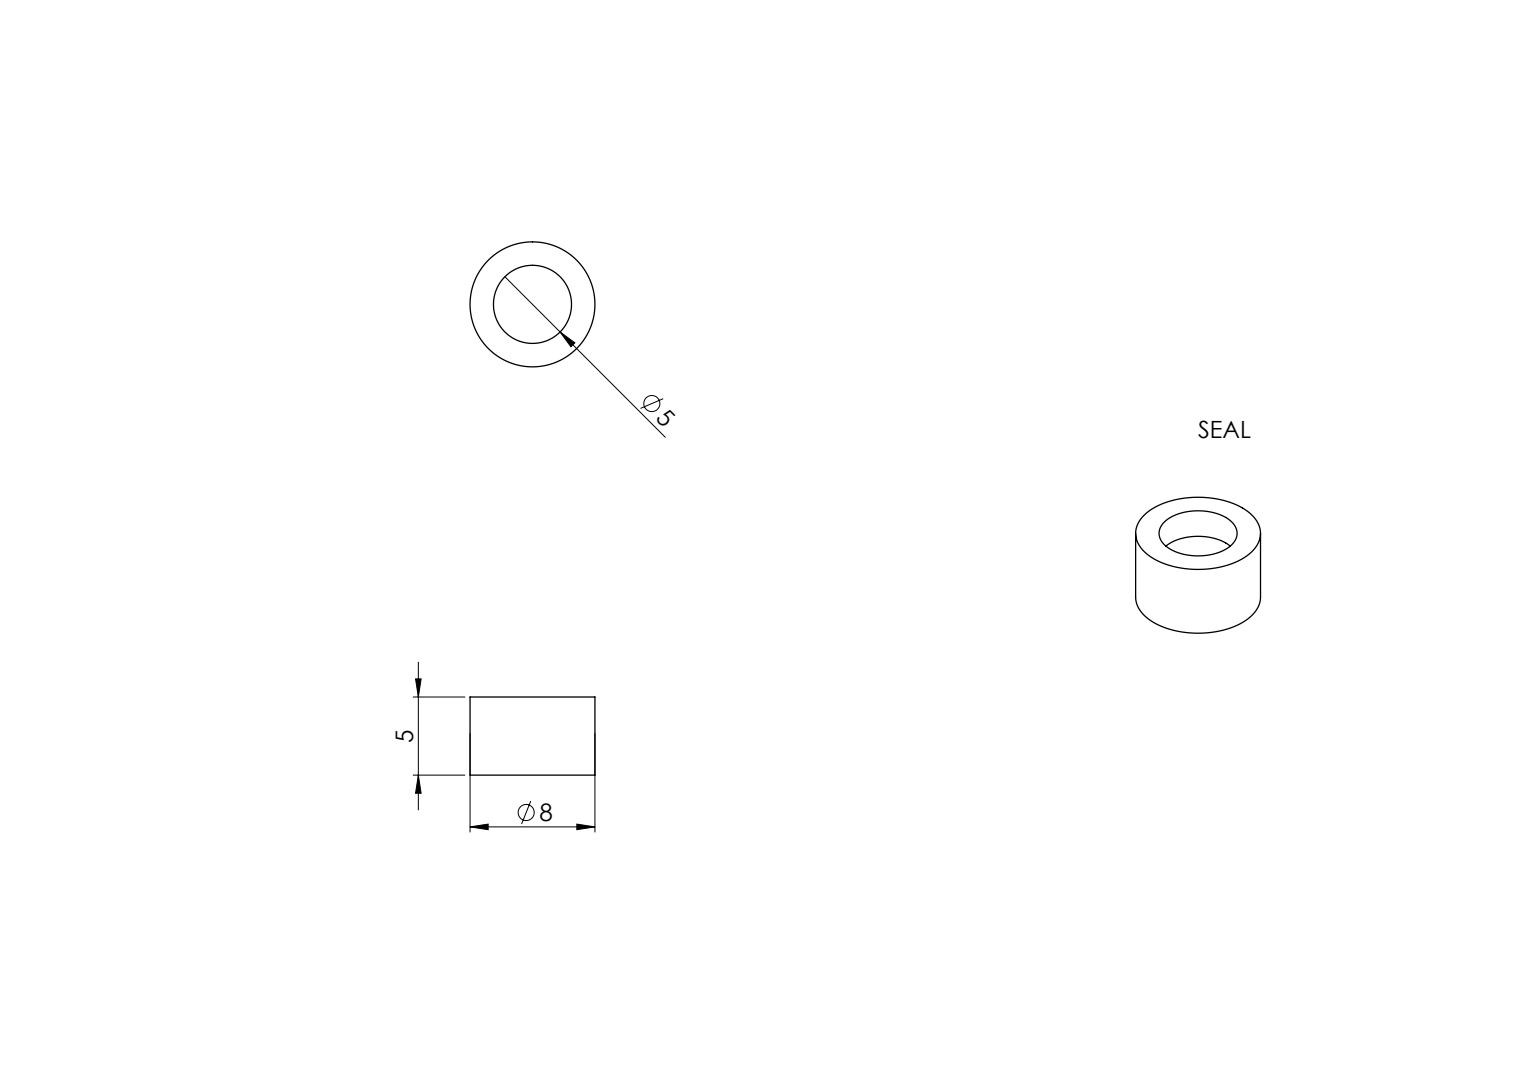
ISO-10303-21;
HEADER;
FILE_DESCRIPTION (('STEP AP214'),
    '1' );
FILE_NAME ('seal.step',
    '2026-10-25T16:39:07',
    ( '' ),
    ( '' ),
    'SwSTEP 2.0',
    'SolidWorks 2026',
    '' );
FILE_SCHEMA (( 'AUTOMOTIVE_DESIGN' ));
ENDSEC;

DATA;
#4=CIRCLE ( 'NONE', #8561, 2.499999999999999556 ) ;
#17=CARTESIAN_POINT ( 'NONE',  ( 0.000000000000000000, 0.000000000000000000, 4.000000000000000000 ) ) ;
#234=CARTESIAN_POINT ( 'NONE',  ( 3.061616997868382648E-16, 3.000000000000000000, -2.499999999999999556 ) ) ;
#340=( GEOMETRIC_REPRESENTATION_CONTEXT ( 3 ) GLOBAL_UNCERTAINTY_ASSIGNED_CONTEXT ( ( #12516 ) ) GLOBAL_UNIT_ASSIGNED_CONTEXT ( ( #1395, #8421, #14269 ) ) REPRESENTATION_CONTEXT ( 'NONE', 'WORKASPACE' ) );
#392=DIRECTION ( 'NONE',  ( 0.000000000000000000, -1.000000000000000000, 0.000000000000000000 ) ) ;
#724=VECTOR ( 'NONE', #10694, 1000.000000000000000 ) ;
#725=PRODUCT_DEFINITION_SHAPE ( 'NONE', 'NONE',  #2104 ) ;
#866=ORIENTED_EDGE ( 'NONE', *, *, #16394, .T. ) ;
#914=AXIS2_PLACEMENT_3D ( 'NONE', #3726, #9376, #2718 ) ;
#1063=DIRECTION ( 'NONE',  ( 0.000000000000000000, -1.000000000000000000, 0.000000000000000000 ) ) ;
#1236=ORIENTED_EDGE ( 'NONE', *, *, #16460, .F. ) ;
#1279=CARTESIAN_POINT ( 'NONE',  ( 0.000000000000000000, 3.000000000000000000, 0.000000000000000000 ) ) ;
#1296=AXIS2_PLACEMENT_3D ( 'NONE', #7926, #9407, #3852 ) ;
#1381=EDGE_CURVE ( 'NONE', #5033, #1782, #14887, .T. ) ;
#1393=FACE_OUTER_BOUND ( 'NONE', #4236, .T. ) ;
#1395=( LENGTH_UNIT ( ) NAMED_UNIT ( * ) SI_UNIT ( .MILLI., .METRE. ) );
#1483=( LENGTH_UNIT ( ) NAMED_UNIT ( * ) SI_UNIT ( .MILLI., .METRE. ) );
#1500=VERTEX_POINT ( 'NONE', #13446 ) ;
#1507=AXIS2_PLACEMENT_3D ( 'NONE', #2357, #6777, #8078 ) ;
#1556=PRODUCT_DEFINITION_FORMATION_WITH_SPECIFIED_SOURCE ( 'ANY', '', #17623, .NOT_KNOWN. ) ;
#1572=PLANE ( 'NONE',  #2737 ) ;
#1586=MANIFOLD_SOLID_BREP ( 'Boss-Extrude2', #14466 ) ;
#1614=CYLINDRICAL_SURFACE ( 'NONE', #16233, 2.499999999999999556 ) ;
#1655=ORIENTED_EDGE ( 'NONE', *, *, #16460, .T. ) ;
#1782=VERTEX_POINT ( 'NONE', #10171 ) ;
#1803=ORIENTED_EDGE ( 'NONE', *, *, #5917, .F. ) ;
#1935=CARTESIAN_POINT ( 'NONE',  ( 0.000000000000000000, 5.000000000000000000, 2.499999999999999556 ) ) ;
#2104=PRODUCT_DEFINITION ( 'UNKNOWN', '', #1556, #14150 ) ;
#2168=STYLED_ITEM('',(#18417),#1586);
#2227=VERTEX_POINT ( 'NONE', #17 ) ;
#2331=LINE ( 'NONE', #12225, #8909 ) ;
#2357=CARTESIAN_POINT ( 'NONE',  ( 0.000000000000000000, 5.000000000000000000, 0.000000000000000000 ) ) ;
#2461=FILL_AREA_STYLE_COLOUR ( '', #10696 ) ;
#2511=ORIENTED_EDGE ( 'NONE', *, *, #16394, .F. ) ;
#2541=CARTESIAN_POINT ( 'NONE',  ( 4.898587196589414801E-16, 0.000000000000000000, -4.000000000000000000 ) ) ;
#2624=DIRECTION ( 'NONE',  ( 0.000000000000000000, 0.000000000000000000, 1.000000000000000000 ) ) ;
#2711=ORIENTED_EDGE ( 'NONE', *, *, #4160, .F. ) ;
#2717=STYLED_ITEM ( 'NONE', ( #12687 ), #5178 ) ;
#2718=DIRECTION ( 'NONE',  ( 0.000000000000000000, 0.000000000000000000, 1.000000000000000000 ) ) ;
#2737=AXIS2_PLACEMENT_3D ( 'NONE', #11659, #7020, #14460 ) ;
#2801=DIRECTION ( 'NONE',  ( 0.000000000000000000, 0.000000000000000000, -1.000000000000000000 ) ) ;
#2957=AXIS2_PLACEMENT_3D ( 'NONE', #8286, #17957, #5417 ) ;
#3271=ADVANCED_FACE ( 'NONE', ( #1393, #15571 ), #1572, .F. ) ;
#3674=DIRECTION ( 'NONE',  ( -0.000000000000000000, 1.000000000000000000, -0.000000000000000000 ) ) ;
#3726=CARTESIAN_POINT ( 'NONE',  ( 0.000000000000000000, 3.000000000000000000, 0.000000000000000000 ) ) ;
#3852=DIRECTION ( 'NONE',  ( 0.000000000000000000, -0.000000000000000000, -1.000000000000000000 ) ) ;
#3895=( LENGTH_UNIT ( ) NAMED_UNIT ( * ) SI_UNIT ( .MILLI., .METRE. ) );
#4160=EDGE_CURVE ( 'NONE', #9997, #1782, #12097, .T. ) ;
#4200=MECHANICAL_DESIGN_GEOMETRIC_PRESENTATION_REPRESENTATION('',(#2717),#13665);
#4231=CYLINDRICAL_SURFACE ( 'NONE', #12756, 4.000000000000001776 ) ;
#4236=EDGE_LOOP ( 'NONE', ( #11681, #1803 ) ) ;
#4258=( NAMED_UNIT ( * ) SI_UNIT ( $, .STERADIAN. ) SOLID_ANGLE_UNIT ( ) );
#4454=CARTESIAN_POINT ( 'NONE',  ( 4.898587196589415787E-16, 5.000000000000000000, -4.000000000000001776 ) ) ;
#4701=LINE ( 'NONE', #15745, #13005 ) ;
#4832=DIRECTION ( 'NONE',  ( 0.000000000000000000, 0.000000000000000000, -1.000000000000000000 ) ) ;
#4912=AXIS2_PLACEMENT_3D ( 'NONE', #12531, #6690, #12344 ) ;
#4946=LINE ( 'NONE', #10601, #724 ) ;
#5033=VERTEX_POINT ( 'NONE', #1935 ) ;
#5058=ORIENTED_EDGE ( 'NONE', *, *, #6349, .T. ) ;
#5113=VECTOR ( 'NONE', #3674, 1000.000000000000000 ) ;
#5178=ADVANCED_BREP_SHAPE_REPRESENTATION ( '', ( #1586, #16940 ), #340 ) ;
#5217=SURFACE_STYLE_USAGE ( .BOTH. , #14175 ) ;
#5244=ADVANCED_FACE ( 'NONE', ( #8020 ), #10805, .T. ) ;
#5417=DIRECTION ( 'NONE',  ( 0.000000000000000000, 0.000000000000000000, -1.000000000000000000 ) ) ;
#5514=ORIENTED_EDGE ( 'NONE', *, *, #16181, .T. ) ;
#5738=CIRCLE ( 'NONE', #10475, 4.000000000000001776 ) ;
#5747=EDGE_CURVE ( 'NONE', #2227, #1500, #4946, .T. ) ;
#5917=EDGE_CURVE ( 'NONE', #12929, #1500, #5738, .T. ) ;
#5944=APPLICATION_CONTEXT ( 'automotive_design' ) ;
#5969=( GEOMETRIC_REPRESENTATION_CONTEXT ( 3 ) GLOBAL_UNCERTAINTY_ASSIGNED_CONTEXT ( ( #6741 ) ) GLOBAL_UNIT_ASSIGNED_CONTEXT ( ( #3895, #8151, #15036 ) ) REPRESENTATION_CONTEXT ( 'NONE', 'WORKASPACE' ) );
#6212=AXIS2_PLACEMENT_3D ( 'NONE', #6625, #12546, #8097 ) ;
#6220=CARTESIAN_POINT ( 'NONE',  ( 0.000000000000000000, 5.000000000000000000, 0.000000000000000000 ) ) ;
#6288=VERTEX_POINT ( 'NONE', #2541 ) ;
#6307=APPLICATION_CONTEXT ( 'automotive_design' ) ;
#6349=EDGE_CURVE ( 'NONE', #15303, #9997, #6975, .T. ) ;
#6428=DIRECTION ( 'NONE',  ( 1.000000000000000000, 0.000000000000000000, 0.000000000000000000 ) ) ;
#6439=CARTESIAN_POINT ( 'NONE',  ( 0.000000000000000000, 3.000000000000000000, 0.000000000000000000 ) ) ;
#6496=ORIENTED_EDGE ( 'NONE', *, *, #1381, .F. ) ;
#6559=ORIENTED_EDGE ( 'NONE', *, *, #5747, .T. ) ;
#6625=CARTESIAN_POINT ( 'NONE',  ( 0.000000000000000000, 5.000000000000000000, 0.000000000000000000 ) ) ;
#6690=DIRECTION ( 'NONE',  ( 0.000000000000000000, -1.000000000000000000, 0.000000000000000000 ) ) ;
#6741=UNCERTAINTY_MEASURE_WITH_UNIT (LENGTH_MEASURE( 1.000000000000000082E-05 ), #3895, 'distance_accuracy_value', 'NONE');
#6777=DIRECTION ( 'NONE',  ( 0.000000000000000000, -1.000000000000000000, 0.000000000000000000 ) ) ;
#6975=CIRCLE ( 'NONE', #4912, 2.499999999999999556 ) ;
#6984=EDGE_LOOP ( 'NONE', ( #18039, #14574, #13989, #15198 ) ) ;
#7020=DIRECTION ( 'NONE',  ( 0.000000000000000000, -1.000000000000000000, 0.000000000000000000 ) ) ;
#7061=CARTESIAN_POINT ( 'NONE',  ( 0.000000000000000000, 3.000000000000000000, 0.000000000000000000 ) ) ;
#7150=CIRCLE ( 'NONE', #14895, 4.000000000000000000 ) ;
#7454=MECHANICAL_DESIGN_GEOMETRIC_PRESENTATION_REPRESENTATION('',(#2168),#5969);
#7745=SHAPE_DEFINITION_REPRESENTATION ( #725, #12769 ) ;
#7838=ORIENTED_EDGE ( 'NONE', *, *, #1381, .T. ) ;
#7926=CARTESIAN_POINT ( 'NONE',  ( 0.000000000000000000, 0.000000000000000000, 0.000000000000000000 ) ) ;
#8020=FACE_OUTER_BOUND ( 'NONE', #12578, .T. ) ;
#8078=DIRECTION ( 'NONE',  ( 0.000000000000000000, 0.000000000000000000, -1.000000000000000000 ) ) ;
#8091=CARTESIAN_POINT ( 'NONE',  ( 0.000000000000000000, 5.000000000000000000, 0.000000000000000000 ) ) ;
#8097=DIRECTION ( 'NONE',  ( 0.000000000000000000, 0.000000000000000000, -1.000000000000000000 ) ) ;
#8143=CARTESIAN_POINT ( 'NONE',  ( 0.000000000000000000, 3.000000000000000000, 2.499999999999999556 ) ) ;
#8151=( NAMED_UNIT ( * ) PLANE_ANGLE_UNIT ( ) SI_UNIT ( $, .RADIAN. ) );
#8169=CYLINDRICAL_SURFACE ( 'NONE', #914, 4.000000000000001776 ) ;
#8177=ORIENTED_EDGE ( 'NONE', *, *, #16181, .F. ) ;
#8286=CARTESIAN_POINT ( 'NONE',  ( 0.000000000000000000, 0.000000000000000000, 0.000000000000000000 ) ) ;
#8325=DIRECTION ( 'NONE',  ( -0.000000000000000000, 1.000000000000000000, -0.000000000000000000 ) ) ;
#8391=EDGE_CURVE ( 'NONE', #6288, #2227, #7150, .T. ) ;
#8421=( NAMED_UNIT ( * ) PLANE_ANGLE_UNIT ( ) SI_UNIT ( $, .RADIAN. ) );
#8561=AXIS2_PLACEMENT_3D ( 'NONE', #6439, #16284, #13393 ) ;
#8711=EDGE_LOOP ( 'NONE', ( #15503, #8177 ) ) ;
#8794=EDGE_CURVE ( 'NONE', #15303, #5033, #2331, .T. ) ;
#8909=VECTOR ( 'NONE', #8325, 1000.000000000000000 ) ;
#9024=CARTESIAN_POINT ( 'NONE',  ( 0.000000000000000000, 0.000000000000000000, 0.000000000000000000 ) ) ;
#9376=DIRECTION ( 'NONE',  ( -0.000000000000000000, 1.000000000000000000, -0.000000000000000000 ) ) ;
#9379=ORIENTED_EDGE ( 'NONE', *, *, #8794, .F. ) ;
#9407=DIRECTION ( 'NONE',  ( 0.000000000000000000, -1.000000000000000000, 0.000000000000000000 ) ) ;
#9540=ORIENTED_EDGE ( 'NONE', *, *, #8794, .T. ) ;
#9722=SURFACE_STYLE_FILL_AREA ( #15662 ) ;
#9807=ORIENTED_EDGE ( 'NONE', *, *, #15615, .F. ) ;
#9901=SHAPE_REPRESENTATION_RELATIONSHIP ( 'NONE' , 'NONE' ,  #12769, #5178 ) ;
#9997=VERTEX_POINT ( 'NONE', #234 ) ;
#10171=CARTESIAN_POINT ( 'NONE',  ( 3.061616997868382648E-16, 5.000000000000000000, -2.499999999999999556 ) ) ;
#10326=ADVANCED_FACE ( 'NONE', ( #11326 ), #10976, .F. ) ;
#10475=AXIS2_PLACEMENT_3D ( 'NONE', #8091, #1063, #13842 ) ;
#10580=AXIS2_PLACEMENT_3D ( 'NONE', #17247, #15324, #2624 ) ;
#10601=CARTESIAN_POINT ( 'NONE',  ( 0.000000000000000000, 3.000000000000000000, 4.000000000000001776 ) ) ;
#10671=CIRCLE ( 'NONE', #1507, 4.000000000000001776 ) ;
#10694=DIRECTION ( 'NONE',  ( -0.000000000000000000, 1.000000000000000000, -0.000000000000000000 ) ) ;
#10696=COLOUR_RGB ( '',0.8941176470588234615, 0.8941176470588234615, 0.8941176470588234615 ) ;
#10709=CARTESIAN_POINT ( 'NONE',  ( 3.061616997868382648E-16, 3.000000000000000000, -2.499999999999999556 ) ) ;
#10787=ADVANCED_FACE ( 'NONE', ( #11555 ), #16636, .F. ) ;
#10805=PLANE ( 'NONE',  #1296 ) ;
#10976=PLANE ( 'NONE',  #12636 ) ;
#11041=DIRECTION ( 'NONE',  ( 0.000000000000000000, -1.000000000000000000, 0.000000000000000000 ) ) ;
#11159=EDGE_LOOP ( 'NONE', ( #2711, #5514, #9540, #2511 ) ) ;
#11247=DIRECTION ( 'NONE',  ( -0.000000000000000000, 1.000000000000000000, -0.000000000000000000 ) ) ;
#11326=FACE_OUTER_BOUND ( 'NONE', #8711, .T. ) ;
#11555=FACE_OUTER_BOUND ( 'NONE', #11159, .T. ) ;
#11659=CARTESIAN_POINT ( 'NONE',  ( 0.000000000000000000, 5.000000000000000000, 0.000000000000000000 ) ) ;
#11665=EDGE_LOOP ( 'NONE', ( #7838, #866 ) ) ;
#11681=ORIENTED_EDGE ( 'NONE', *, *, #17049, .F. ) ;
#12097=LINE ( 'NONE', #10709, #5113 ) ;
#12225=CARTESIAN_POINT ( 'NONE',  ( 0.000000000000000000, 3.000000000000000000, 2.499999999999999556 ) ) ;
#12344=DIRECTION ( 'NONE',  ( 0.000000000000000000, 0.000000000000000000, -1.000000000000000000 ) ) ;
#12390=DIRECTION ( 'NONE',  ( -0.000000000000000000, 1.000000000000000000, -0.000000000000000000 ) ) ;
#12516=UNCERTAINTY_MEASURE_WITH_UNIT (LENGTH_MEASURE( 1.000000000000000082E-05 ), #1395, 'distance_accuracy_value', 'NONE');
#12531=CARTESIAN_POINT ( 'NONE',  ( 0.000000000000000000, 3.000000000000000000, 0.000000000000000000 ) ) ;
#12546=DIRECTION ( 'NONE',  ( 0.000000000000000000, -1.000000000000000000, 0.000000000000000000 ) ) ;
#12578=EDGE_LOOP ( 'NONE', ( #1655, #17930 ) ) ;
#12636=AXIS2_PLACEMENT_3D ( 'NONE', #7061, #18322, #14216 ) ;
#12639=CARTESIAN_POINT ( 'NONE',  ( 0.000000000000000000, 3.000000000000000000, 0.000000000000000000 ) ) ;
#12687=PRESENTATION_STYLE_ASSIGNMENT (( #5217 ) ) ;
#12730=CIRCLE ( 'NONE', #6212, 2.499999999999999556 ) ;
#12756=AXIS2_PLACEMENT_3D ( 'NONE', #1279, #12390, #15549 ) ;
#12769=SHAPE_REPRESENTATION ( 'seal', ( #16940 ), #340 ) ;
#12929=VERTEX_POINT ( 'NONE', #4454 ) ;
#13005=VECTOR ( 'NONE', #17246, 1000.000000000000000 ) ;
#13393=DIRECTION ( 'NONE',  ( 0.000000000000000000, 0.000000000000000000, -1.000000000000000000 ) ) ;
#13446=CARTESIAN_POINT ( 'NONE',  ( 0.000000000000000000, 5.000000000000000000, 4.000000000000001776 ) ) ;
#13557=DIRECTION ( 'NONE',  ( 0.000000000000000000, 0.000000000000000000, 1.000000000000000000 ) ) ;
#13580=PRODUCT_CONTEXT ( 'NONE', #5944, 'mechanical' ) ;
#13665=( GEOMETRIC_REPRESENTATION_CONTEXT ( 3 ) GLOBAL_UNCERTAINTY_ASSIGNED_CONTEXT ( ( #16807 ) ) GLOBAL_UNIT_ASSIGNED_CONTEXT ( ( #1483, #16981, #4258 ) ) REPRESENTATION_CONTEXT ( 'NONE', 'WORKASPACE' ) );
#13772=ADVANCED_FACE ( 'NONE', ( #18328 ), #1614, .F. ) ;
#13842=DIRECTION ( 'NONE',  ( 0.000000000000000000, 0.000000000000000000, -1.000000000000000000 ) ) ;
#13989=ORIENTED_EDGE ( 'NONE', *, *, #5917, .T. ) ;
#14150=PRODUCT_DEFINITION_CONTEXT ( 'detailed design', #6307, 'design' ) ;
#14175=SURFACE_SIDE_STYLE ('',( #9722 ) ) ;
#14216=DIRECTION ( 'NONE',  ( 0.000000000000000000, -0.000000000000000000, -1.000000000000000000 ) ) ;
#14269=( NAMED_UNIT ( * ) SI_UNIT ( $, .STERADIAN. ) SOLID_ANGLE_UNIT ( ) );
#14460=DIRECTION ( 'NONE',  ( 0.000000000000000000, -0.000000000000000000, -1.000000000000000000 ) ) ;
#14466=CLOSED_SHELL ( 'NONE', ( #13772, #17730, #3271, #17096, #10787, #10326, #5244 ) ) ;
#14505=EDGE_LOOP ( 'NONE', ( #5058, #16433, #6496, #9379 ) ) ;
#14574=ORIENTED_EDGE ( 'NONE', *, *, #15615, .T. ) ;
#14887=CIRCLE ( 'NONE', #15180, 2.499999999999999556 ) ;
#14895=AXIS2_PLACEMENT_3D ( 'NONE', #16634, #11041, #2801 ) ;
#15036=( NAMED_UNIT ( * ) SI_UNIT ( $, .STERADIAN. ) SOLID_ANGLE_UNIT ( ) );
#15180=AXIS2_PLACEMENT_3D ( 'NONE', #6220, #392, #4832 ) ;
#15198=ORIENTED_EDGE ( 'NONE', *, *, #5747, .F. ) ;
#15241=FACE_OUTER_BOUND ( 'NONE', #17072, .T. ) ;
#15303=VERTEX_POINT ( 'NONE', #8143 ) ;
#15324=DIRECTION ( 'NONE',  ( -0.000000000000000000, 1.000000000000000000, -0.000000000000000000 ) ) ;
#15375=FACE_OUTER_BOUND ( 'NONE', #6984, .T. ) ;
#15503=ORIENTED_EDGE ( 'NONE', *, *, #6349, .F. ) ;
#15549=DIRECTION ( 'NONE',  ( 0.000000000000000000, 0.000000000000000000, 1.000000000000000000 ) ) ;
#15571=FACE_BOUND ( 'NONE', #11665, .T. ) ;
#15615=EDGE_CURVE ( 'NONE', #6288, #12929, #4701, .T. ) ;
#15662=FILL_AREA_STYLE ('',( #2461 ) ) ;
#15745=CARTESIAN_POINT ( 'NONE',  ( 4.898587196589415787E-16, 3.000000000000000000, -4.000000000000001776 ) ) ;
#16181=EDGE_CURVE ( 'NONE', #9997, #15303, #4, .T. ) ;
#16233=AXIS2_PLACEMENT_3D ( 'NONE', #12639, #11247, #17025 ) ;
#16284=DIRECTION ( 'NONE',  ( 0.000000000000000000, -1.000000000000000000, 0.000000000000000000 ) ) ;
#16394=EDGE_CURVE ( 'NONE', #1782, #5033, #12730, .T. ) ;
#16433=ORIENTED_EDGE ( 'NONE', *, *, #4160, .T. ) ;
#16460=EDGE_CURVE ( 'NONE', #2227, #6288, #16595, .T. ) ;
#16593=ORIENTED_EDGE ( 'NONE', *, *, #17049, .T. ) ;
#16595=CIRCLE ( 'NONE', #2957, 4.000000000000000000 ) ;
#16634=CARTESIAN_POINT ( 'NONE',  ( 0.000000000000000000, 0.000000000000000000, 0.000000000000000000 ) ) ;
#16636=CYLINDRICAL_SURFACE ( 'NONE', #10580, 2.499999999999999556 ) ;
#16807=UNCERTAINTY_MEASURE_WITH_UNIT (LENGTH_MEASURE( 1.000000000000000082E-05 ), #1483, 'distance_accuracy_value', 'NONE');
#16940=AXIS2_PLACEMENT_3D ( 'NONE', #9024, #13557, #6428 ) ;
#16981=( NAMED_UNIT ( * ) PLANE_ANGLE_UNIT ( ) SI_UNIT ( $, .RADIAN. ) );
#17025=DIRECTION ( 'NONE',  ( 0.000000000000000000, 0.000000000000000000, 1.000000000000000000 ) ) ;
#17049=EDGE_CURVE ( 'NONE', #1500, #12929, #10671, .T. ) ;
#17072=EDGE_LOOP ( 'NONE', ( #9807, #1236, #6559, #16593 ) ) ;
#17096=ADVANCED_FACE ( 'NONE', ( #15241 ), #8169, .T. ) ;
#17246=DIRECTION ( 'NONE',  ( -0.000000000000000000, 1.000000000000000000, -0.000000000000000000 ) ) ;
#17247=CARTESIAN_POINT ( 'NONE',  ( 0.000000000000000000, 3.000000000000000000, 0.000000000000000000 ) ) ;
#17623=PRODUCT ( 'seal', 'seal', '', ( #13580 ) ) ;
#17730=ADVANCED_FACE ( 'NONE', ( #15375 ), #4231, .T. ) ;
#17930=ORIENTED_EDGE ( 'NONE', *, *, #8391, .T. ) ;
#17957=DIRECTION ( 'NONE',  ( 0.000000000000000000, -1.000000000000000000, 0.000000000000000000 ) ) ;
#18039=ORIENTED_EDGE ( 'NONE', *, *, #8391, .F. ) ;
#18322=DIRECTION ( 'NONE',  ( 0.000000000000000000, -1.000000000000000000, 0.000000000000000000 ) ) ;
#18328=FACE_OUTER_BOUND ( 'NONE', #14505, .T. ) ;
#18411=COLOUR_RGB('Black',0.12,0.14,0.17);
#18412=FILL_AREA_STYLE_COLOUR('',#18411);
#18413=FILL_AREA_STYLE('',(#18412));
#18414=SURFACE_STYLE_FILL_AREA(#18413);
#18415=SURFACE_SIDE_STYLE('',(#18414));
#18416=SURFACE_STYLE_USAGE(.BOTH.,#18415);
#18417=PRESENTATION_STYLE_ASSIGNMENT((#18416));
ENDSEC;
END-ISO-10303-21;
